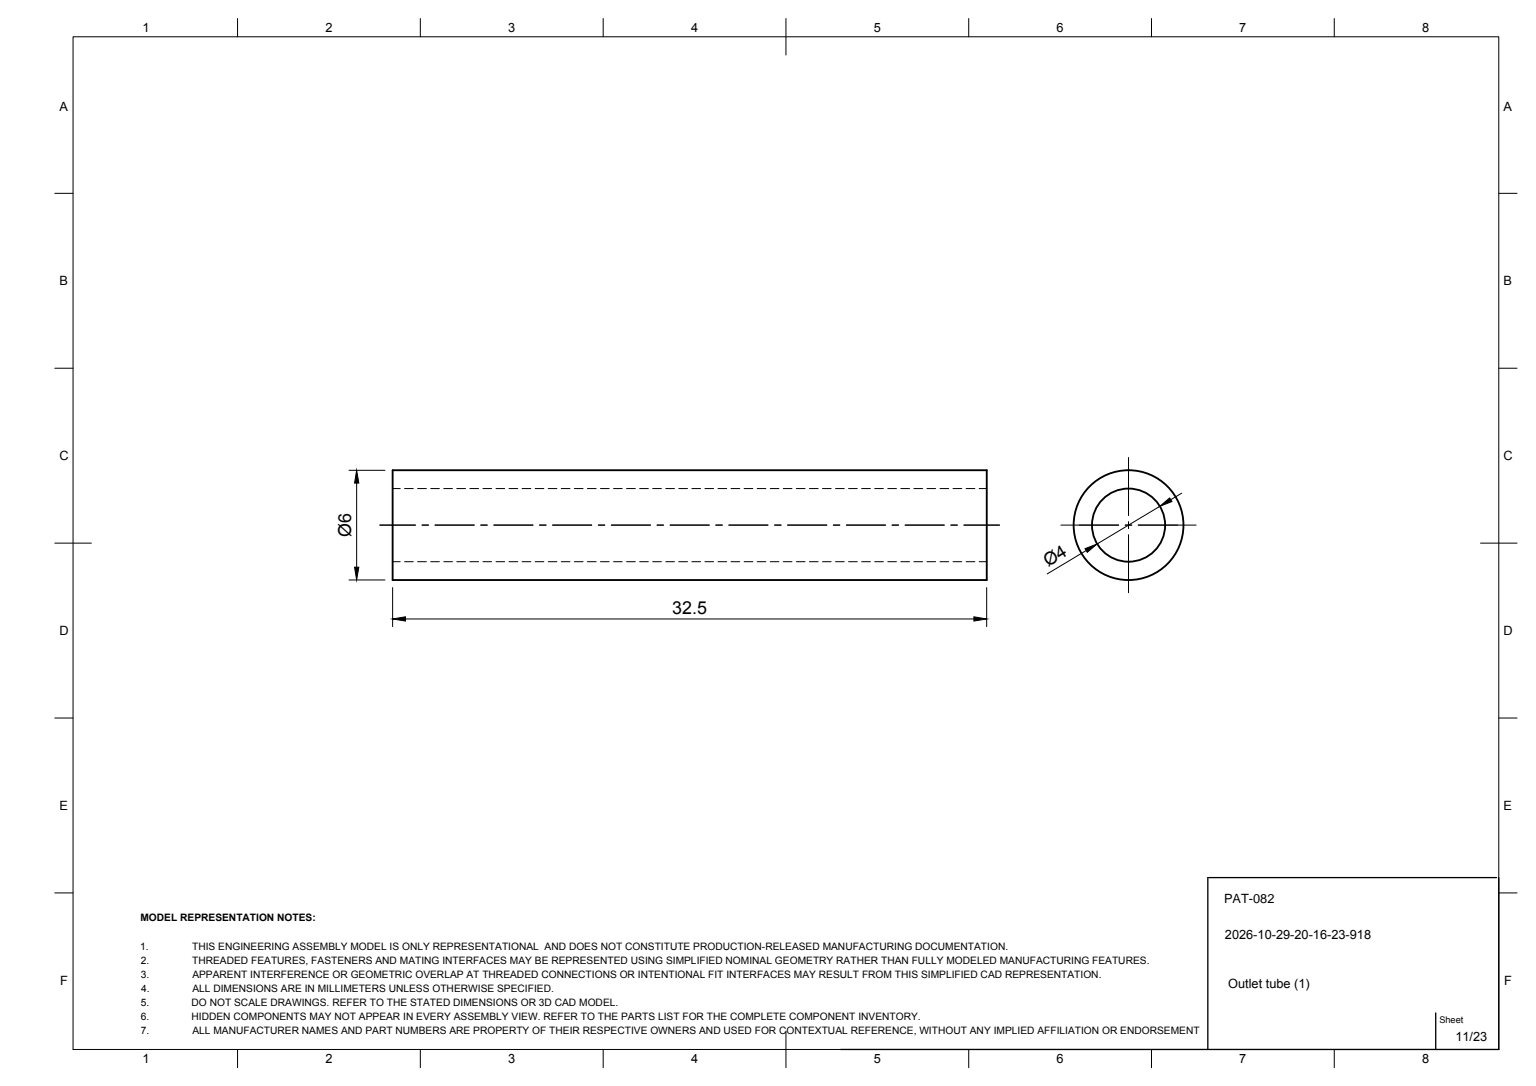
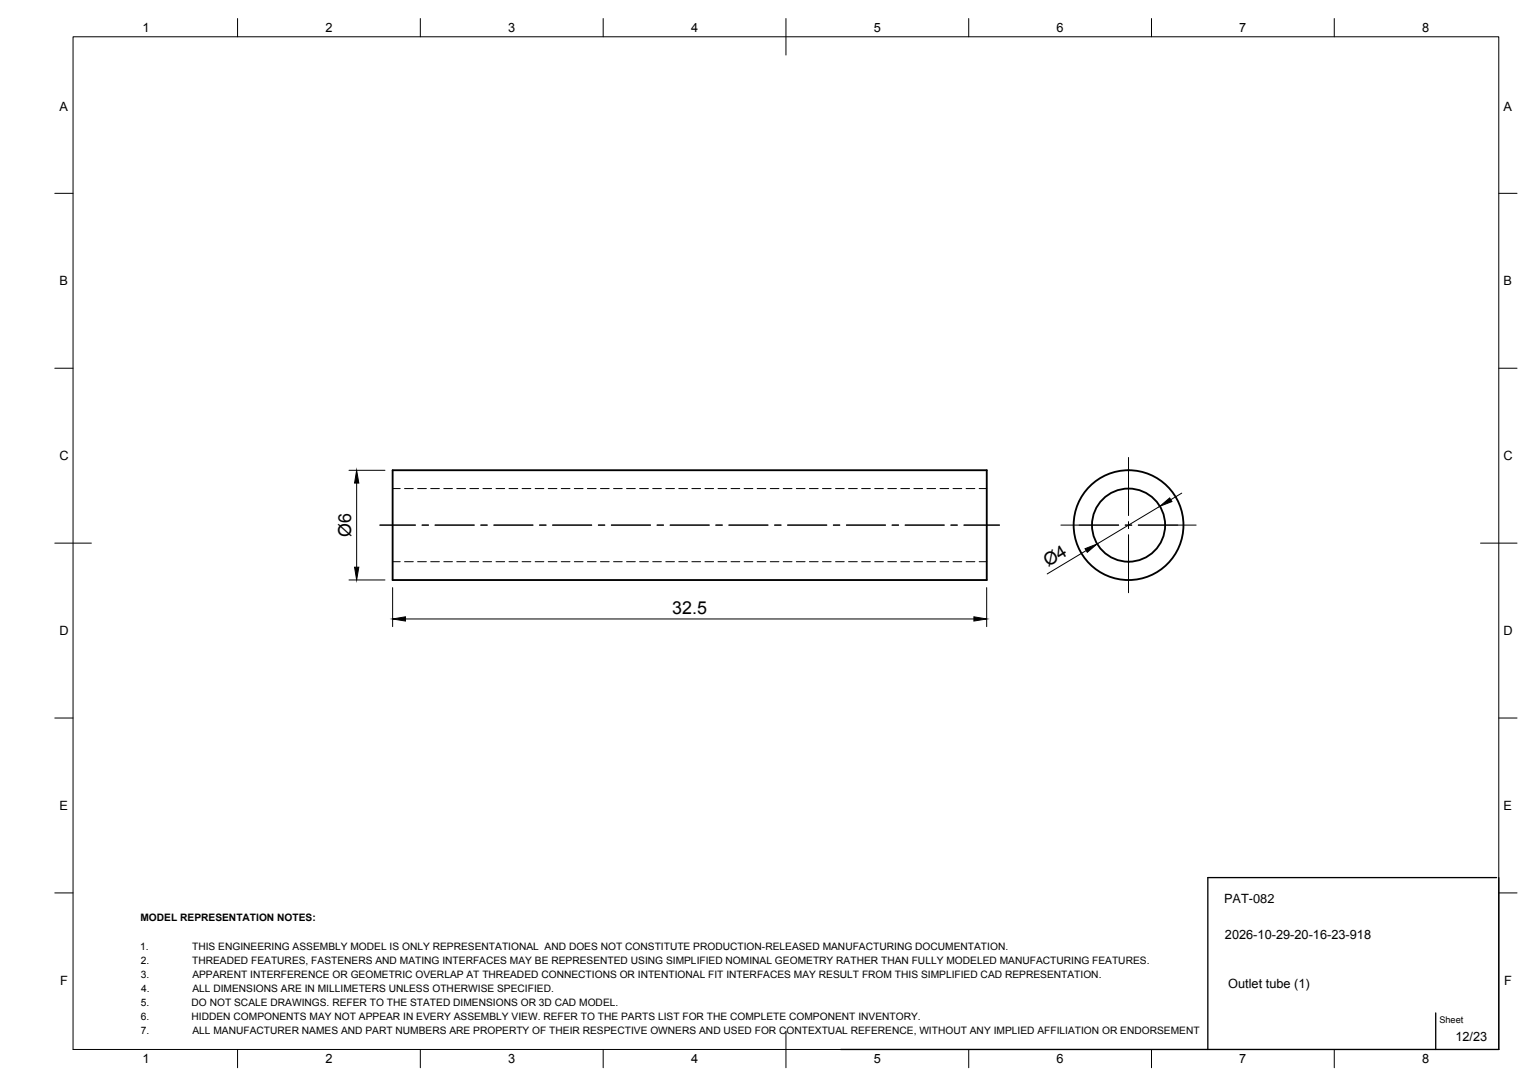
ISO-10303-21;
HEADER;
/* Generated by software containing ST-Developer
 * from STEP Tools, Inc. (www.steptools.com) 
 */

FILE_DESCRIPTION(
/* description */ ('PAT-082'),
/* implementation_level */ '2;1');

FILE_NAME(
/* name */ 'Outlet tube (1).step',
/* time_stamp */ '2026-10-29T20:16:13-07:00',
/* author */ (''),
/* organization */ (''),
/* preprocessor_version */ 'ST-DEVELOPER v20.2',
/* originating_system */ 'Autodesk Translation Framework v15.17.0.0',
/* authorisation */ '');

FILE_SCHEMA (('AUTOMOTIVE_DESIGN { 1 0 10303 214 3 1 1 }'));
ENDSEC;

DATA;
#10=MECHANICAL_DESIGN_GEOMETRIC_PRESENTATION_REPRESENTATION('',(#250),#8266);
#206=SHAPE_REPRESENTATION_RELATIONSHIP('SRR','None',#8368,#228);
#228=ADVANCED_BREP_SHAPE_REPRESENTATION('',(#272),#8252);
#250=STYLED_ITEM('',(#8530),#272);
#272=MANIFOLD_SOLID_BREP('Body1',#4590);
#378=FACE_BOUND('',#1088,.T.);
#379=FACE_BOUND('',#1090,.T.);
#489=PLANE('',#5145);
#490=PLANE('',#5146);
#719=FACE_OUTER_BOUND('',#1085,.T.);
#720=FACE_OUTER_BOUND('',#1086,.T.);
#721=FACE_OUTER_BOUND('',#1087,.T.);
#722=FACE_OUTER_BOUND('',#1089,.T.);
#1085=EDGE_LOOP('',(#3764,#3765,#3766,#3767));
#1086=EDGE_LOOP('',(#3768,#3769,#3770,#3771));
#1087=EDGE_LOOP('',(#3772));
#1088=EDGE_LOOP('',(#3773));
#1089=EDGE_LOOP('',(#3774));
#1090=EDGE_LOOP('',(#3775));
#1430=LINE('',#7670,#1785);
#1431=LINE('',#7676,#1786);
#1785=VECTOR('',#6161,0.2);
#1786=VECTOR('',#6168,0.3);
#2077=CIRCLE('',#5140,0.2);
#2078=CIRCLE('',#5141,0.2);
#2079=CIRCLE('',#5143,0.3);
#2080=CIRCLE('',#5144,0.3);
#2371=VERTEX_POINT('',#7667);
#2372=VERTEX_POINT('',#7669);
#2373=VERTEX_POINT('',#7673);
#2374=VERTEX_POINT('',#7675);
#2858=EDGE_CURVE('',#2371,#2371,#2077,.T.);
#2859=EDGE_CURVE('',#2371,#2372,#1430,.T.);
#2860=EDGE_CURVE('',#2372,#2372,#2078,.T.);
#2861=EDGE_CURVE('',#2373,#2373,#2079,.T.);
#2862=EDGE_CURVE('',#2373,#2374,#1431,.T.);
#2863=EDGE_CURVE('',#2374,#2374,#2080,.T.);
#3764=ORIENTED_EDGE('',*,*,#2858,.F.);
#3765=ORIENTED_EDGE('',*,*,#2859,.T.);
#3766=ORIENTED_EDGE('',*,*,#2860,.T.);
#3767=ORIENTED_EDGE('',*,*,#2859,.F.);
#3768=ORIENTED_EDGE('',*,*,#2861,.F.);
#3769=ORIENTED_EDGE('',*,*,#2862,.T.);
#3770=ORIENTED_EDGE('',*,*,#2863,.T.);
#3771=ORIENTED_EDGE('',*,*,#2862,.F.);
#3772=ORIENTED_EDGE('',*,*,#2861,.T.);
#3773=ORIENTED_EDGE('',*,*,#2858,.T.);
#3774=ORIENTED_EDGE('',*,*,#2863,.F.);
#3775=ORIENTED_EDGE('',*,*,#2860,.F.);
#4283=CYLINDRICAL_SURFACE('',#5139,0.2);
#4284=CYLINDRICAL_SURFACE('',#5142,0.3);
#4458=ADVANCED_FACE('',(#719),#4283,.F.);
#4459=ADVANCED_FACE('',(#720),#4284,.T.);
#4460=ADVANCED_FACE('',(#721,#378),#489,.T.);
#4461=ADVANCED_FACE('',(#722,#379),#490,.F.);
#4590=CLOSED_SHELL('',(#4458,#4459,#4460,#4461));
#5138=AXIS2_PLACEMENT_3D('',#7665,#6155,#6156);
#5139=AXIS2_PLACEMENT_3D('',#7666,#6157,#6158);
#5140=AXIS2_PLACEMENT_3D('',#7668,#6159,#6160);
#5141=AXIS2_PLACEMENT_3D('',#7671,#6162,#6163);
#5142=AXIS2_PLACEMENT_3D('',#7672,#6164,#6165);
#5143=AXIS2_PLACEMENT_3D('',#7674,#6166,#6167);
#5144=AXIS2_PLACEMENT_3D('',#7677,#6169,#6170);
#5145=AXIS2_PLACEMENT_3D('',#7678,#6171,#6172);
#5146=AXIS2_PLACEMENT_3D('',#7679,#6173,#6174);
#6155=DIRECTION('axis',(0.,0.,1.));
#6156=DIRECTION('refdir',(1.,0.,0.));
#6157=DIRECTION('center_axis',(0.,0.,1.));
#6158=DIRECTION('ref_axis',(1.,0.,0.));
#6159=DIRECTION('center_axis',(0.,0.,-1.));
#6160=DIRECTION('ref_axis',(1.,0.,0.));
#6161=DIRECTION('',(0.,0.,-1.));
#6162=DIRECTION('center_axis',(0.,0.,-1.));
#6163=DIRECTION('ref_axis',(1.,0.,0.));
#6164=DIRECTION('center_axis',(0.,0.,1.));
#6165=DIRECTION('ref_axis',(1.,0.,0.));
#6166=DIRECTION('center_axis',(0.,0.,1.));
#6167=DIRECTION('ref_axis',(1.,0.,0.));
#6168=DIRECTION('',(0.,0.,-1.));
#6169=DIRECTION('center_axis',(0.,0.,1.));
#6170=DIRECTION('ref_axis',(1.,0.,0.));
#6171=DIRECTION('center_axis',(0.,0.,1.));
#6172=DIRECTION('ref_axis',(1.,0.,0.));
#6173=DIRECTION('center_axis',(0.,0.,1.));
#6174=DIRECTION('ref_axis',(1.,0.,0.));
#7665=CARTESIAN_POINT('',(0.,0.,0.));
#7666=CARTESIAN_POINT('Origin',(-1.25,0.,5.7));
#7667=CARTESIAN_POINT('',(-1.45,-2.44929359829471E-17,8.95));
#7668=CARTESIAN_POINT('Origin',(-1.25,0.,8.95));
#7669=CARTESIAN_POINT('',(-1.45,-2.44929359829471E-17,5.7));
#7670=CARTESIAN_POINT('',(-1.45,-2.44929359829471E-17,5.7));
#7671=CARTESIAN_POINT('Origin',(-1.25,0.,5.7));
#7672=CARTESIAN_POINT('Origin',(-1.25,0.,5.7));
#7673=CARTESIAN_POINT('',(-1.55,-3.67394039744206E-17,8.95));
#7674=CARTESIAN_POINT('Origin',(-1.25,0.,8.95));
#7675=CARTESIAN_POINT('',(-1.55,-3.67394039744206E-17,5.7));
#7676=CARTESIAN_POINT('',(-1.55,-3.67394039744206E-17,5.7));
#7677=CARTESIAN_POINT('Origin',(-1.25,0.,5.7));
#7678=CARTESIAN_POINT('Origin',(-1.25,0.,8.95));
#7679=CARTESIAN_POINT('Origin',(-1.25,0.,5.7));
#8227=UNCERTAINTY_MEASURE_WITH_UNIT(LENGTH_MEASURE(0.001),#8267,
'DISTANCE_ACCURACY_VALUE',
'Maximum model space distance between geometric entities at asserted c
onnectivities');
#8241=UNCERTAINTY_MEASURE_WITH_UNIT(LENGTH_MEASURE(0.001),#8267,
'DISTANCE_ACCURACY_VALUE',
'Maximum model space distance between geometric entities at asserted c
onnectivities');
#8252=(
GEOMETRIC_REPRESENTATION_CONTEXT(3)
GLOBAL_UNCERTAINTY_ASSIGNED_CONTEXT((#8227))
GLOBAL_UNIT_ASSIGNED_CONTEXT((#8267,#8269,#8270))
REPRESENTATION_CONTEXT('','3D')
);
#8266=(
GEOMETRIC_REPRESENTATION_CONTEXT(3)
GLOBAL_UNCERTAINTY_ASSIGNED_CONTEXT((#8241))
GLOBAL_UNIT_ASSIGNED_CONTEXT((#8267,#8269,#8270))
REPRESENTATION_CONTEXT('','3D')
);
#8267=(
LENGTH_UNIT()
NAMED_UNIT(*)
SI_UNIT(.CENTI.,.METRE.)
);
#8269=(
NAMED_UNIT(*)
PLANE_ANGLE_UNIT()
SI_UNIT($,.RADIAN.)
);
#8270=(
NAMED_UNIT(*)
SI_UNIT($,.STERADIAN.)
SOLID_ANGLE_UNIT()
);
#8281=SHAPE_DEFINITION_REPRESENTATION(#8305,#8368);
#8305=PRODUCT_DEFINITION_SHAPE('',$,#8393);
#8368=SHAPE_REPRESENTATION('',(#5138),#8252);
#8382=PRODUCT_DEFINITION_CONTEXT('part definition',#8456,'design');
#8393=PRODUCT_DEFINITION('Outlet tube (1)','Outlet tube (1)',
#8417,#8382);
#8417=PRODUCT_DEFINITION_FORMATION('',$,#8468);
#8456=APPLICATION_CONTEXT(
'Core Data for Automotive Mechanical Design Process');
#8457=PRODUCT_CONTEXT('part definition',#8456,'mechanical');
#8468=PRODUCT('Outlet tube (1)','Outlet tube (1)',
'Outlet tube (1)',(#8457));
#8524=COLOUR_RGB('Sky Blue',0.24,0.69,0.87);
#8525=FILL_AREA_STYLE_COLOUR('',#8524);
#8526=FILL_AREA_STYLE('',(#8525));
#8527=SURFACE_STYLE_FILL_AREA(#8526);
#8528=SURFACE_SIDE_STYLE('',(#8527));
#8529=SURFACE_STYLE_USAGE(.BOTH.,#8528);
#8530=PRESENTATION_STYLE_ASSIGNMENT((#8529));
ENDSEC;
END-ISO-10303-21;
